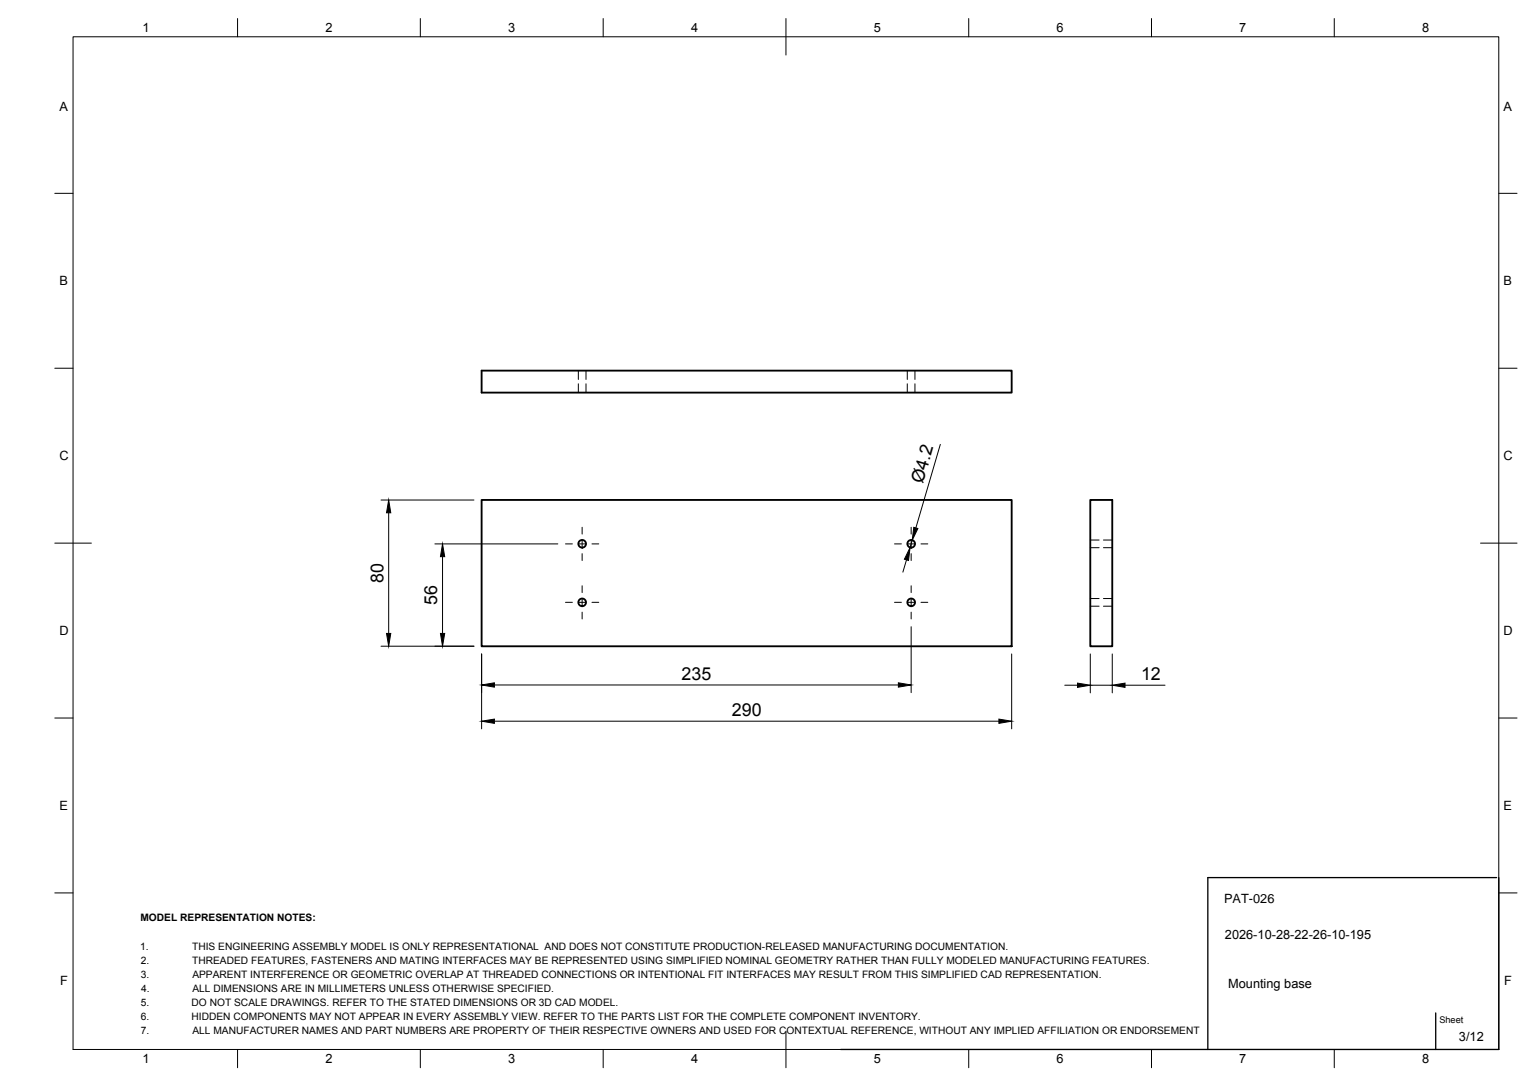
ISO-10303-21;
HEADER;
/* Generated by software containing ST-Developer
 * from STEP Tools, Inc. (www.steptools.com) 
 */

FILE_DESCRIPTION(
/* description */ ('PAT-026'),
/* implementation_level */ '2;1');

FILE_NAME(
/* name */ 'Mounting base.step',
/* time_stamp */ '2026-10-28T22:25:58-07:00',
/* author */ (''),
/* organization */ (''),
/* preprocessor_version */ 'ST-DEVELOPER v20.2',
/* originating_system */ 'Autodesk Translation Framework v15.17.0.0',
/* authorisation */ '');

FILE_SCHEMA (('AUTOMOTIVE_DESIGN { 1 0 10303 214 3 1 1 }'));
ENDSEC;

DATA;
#10=MECHANICAL_DESIGN_GEOMETRIC_PRESENTATION_REPRESENTATION('',(#141),#12343);
#119=SHAPE_REPRESENTATION_RELATIONSHIP('SRR','None',#12396,#130);
#130=ADVANCED_BREP_SHAPE_REPRESENTATION('',(#152),#12331);
#141=STYLED_ITEM('',(#12512),#152);
#152=MANIFOLD_SOLID_BREP('Body1',#7347);
#161=FACE_BOUND('',#965,.T.);
#162=FACE_BOUND('',#966,.T.);
#163=FACE_BOUND('',#967,.T.);
#164=FACE_BOUND('',#968,.T.);
#165=FACE_BOUND('',#970,.T.);
#166=FACE_BOUND('',#971,.T.);
#167=FACE_BOUND('',#972,.T.);
#168=FACE_BOUND('',#973,.T.);
#194=PLANE('',#7496);
#195=PLANE('',#7497);
#196=PLANE('',#7498);
#197=PLANE('',#7499);
#198=PLANE('',#7500);
#199=PLANE('',#7501);
#553=FACE_OUTER_BOUND('',#956,.T.);
#554=FACE_OUTER_BOUND('',#957,.T.);
#555=FACE_OUTER_BOUND('',#958,.T.);
#556=FACE_OUTER_BOUND('',#959,.T.);
#557=FACE_OUTER_BOUND('',#960,.T.);
#558=FACE_OUTER_BOUND('',#961,.T.);
#559=FACE_OUTER_BOUND('',#962,.T.);
#560=FACE_OUTER_BOUND('',#963,.T.);
#561=FACE_OUTER_BOUND('',#964,.T.);
#562=FACE_OUTER_BOUND('',#969,.T.);
#956=EDGE_LOOP('',(#4899,#4900,#4901,#4902));
#957=EDGE_LOOP('',(#4903,#4904,#4905,#4906));
#958=EDGE_LOOP('',(#4907,#4908,#4909,#4910));
#959=EDGE_LOOP('',(#4911,#4912,#4913,#4914));
#960=EDGE_LOOP('',(#4915,#4916,#4917,#4918));
#961=EDGE_LOOP('',(#4919,#4920,#4921,#4922));
#962=EDGE_LOOP('',(#4923,#4924,#4925,#4926));
#963=EDGE_LOOP('',(#4927,#4928,#4929,#4930));
#964=EDGE_LOOP('',(#4931,#4932,#4933,#4934));
#965=EDGE_LOOP('',(#4935));
#966=EDGE_LOOP('',(#4936));
#967=EDGE_LOOP('',(#4937));
#968=EDGE_LOOP('',(#4938));
#969=EDGE_LOOP('',(#4939,#4940,#4941,#4942));
#970=EDGE_LOOP('',(#4943));
#971=EDGE_LOOP('',(#4944));
#972=EDGE_LOOP('',(#4945));
#973=EDGE_LOOP('',(#4946));
#1392=LINE('',#10046,#2264);
#1393=LINE('',#10052,#2265);
#1394=LINE('',#10058,#2266);
#1395=LINE('',#10064,#2267);
#1396=LINE('',#10069,#2268);
#1397=LINE('',#10071,#2269);
#1398=LINE('',#10073,#2270);
#1399=LINE('',#10074,#2271);
#1400=LINE('',#10077,#2272);
#1401=LINE('',#10079,#2273);
#1402=LINE('',#10080,#2274);
#1403=LINE('',#10083,#2275);
#1404=LINE('',#10085,#2276);
#1405=LINE('',#10086,#2277);
#1406=LINE('',#10088,#2278);
#1407=LINE('',#10089,#2279);
#2264=VECTOR('',#8052,0.21);
#2265=VECTOR('',#8059,0.21);
#2266=VECTOR('',#8066,0.21);
#2267=VECTOR('',#8073,0.21);
#2268=VECTOR('',#8078,1.);
#2269=VECTOR('',#8079,1.);
#2270=VECTOR('',#8080,1.);
#2271=VECTOR('',#8081,1.);
#2272=VECTOR('',#8084,1.);
#2273=VECTOR('',#8085,1.);
#2274=VECTOR('',#8086,1.);
#2275=VECTOR('',#8089,1.);
#2276=VECTOR('',#8090,1.);
#2277=VECTOR('',#8091,1.);
#2278=VECTOR('',#8094,1.);
#2279=VECTOR('',#8095,1.);
#3136=CIRCLE('',#7485,0.21);
#3137=CIRCLE('',#7486,0.21);
#3138=CIRCLE('',#7488,0.21);
#3139=CIRCLE('',#7489,0.21);
#3140=CIRCLE('',#7491,0.21);
#3141=CIRCLE('',#7492,0.21);
#3142=CIRCLE('',#7494,0.21);
#3143=CIRCLE('',#7495,0.21);
#3261=VERTEX_POINT('',#10043);
#3262=VERTEX_POINT('',#10045);
#3263=VERTEX_POINT('',#10049);
#3264=VERTEX_POINT('',#10051);
#3265=VERTEX_POINT('',#10055);
#3266=VERTEX_POINT('',#10057);
#3267=VERTEX_POINT('',#10061);
#3268=VERTEX_POINT('',#10063);
#3269=VERTEX_POINT('',#10067);
#3270=VERTEX_POINT('',#10068);
#3271=VERTEX_POINT('',#10070);
#3272=VERTEX_POINT('',#10072);
#3273=VERTEX_POINT('',#10076);
#3274=VERTEX_POINT('',#10078);
#3275=VERTEX_POINT('',#10082);
#3276=VERTEX_POINT('',#10084);
#3893=EDGE_CURVE('',#3261,#3261,#3136,.T.);
#3894=EDGE_CURVE('',#3261,#3262,#1392,.T.);
#3895=EDGE_CURVE('',#3262,#3262,#3137,.T.);
#3896=EDGE_CURVE('',#3263,#3263,#3138,.T.);
#3897=EDGE_CURVE('',#3263,#3264,#1393,.T.);
#3898=EDGE_CURVE('',#3264,#3264,#3139,.T.);
#3899=EDGE_CURVE('',#3265,#3265,#3140,.T.);
#3900=EDGE_CURVE('',#3265,#3266,#1394,.T.);
#3901=EDGE_CURVE('',#3266,#3266,#3141,.T.);
#3902=EDGE_CURVE('',#3267,#3267,#3142,.T.);
#3903=EDGE_CURVE('',#3267,#3268,#1395,.T.);
#3904=EDGE_CURVE('',#3268,#3268,#3143,.T.);
#3905=EDGE_CURVE('',#3269,#3270,#1396,.T.);
#3906=EDGE_CURVE('',#3270,#3271,#1397,.T.);
#3907=EDGE_CURVE('',#3272,#3271,#1398,.T.);
#3908=EDGE_CURVE('',#3269,#3272,#1399,.T.);
#3909=EDGE_CURVE('',#3273,#3269,#1400,.T.);
#3910=EDGE_CURVE('',#3274,#3272,#1401,.T.);
#3911=EDGE_CURVE('',#3273,#3274,#1402,.T.);
#3912=EDGE_CURVE('',#3275,#3273,#1403,.T.);
#3913=EDGE_CURVE('',#3276,#3274,#1404,.T.);
#3914=EDGE_CURVE('',#3275,#3276,#1405,.T.);
#3915=EDGE_CURVE('',#3270,#3275,#1406,.T.);
#3916=EDGE_CURVE('',#3271,#3276,#1407,.T.);
#4899=ORIENTED_EDGE('',*,*,#3893,.F.);
#4900=ORIENTED_EDGE('',*,*,#3894,.T.);
#4901=ORIENTED_EDGE('',*,*,#3895,.F.);
#4902=ORIENTED_EDGE('',*,*,#3894,.F.);
#4903=ORIENTED_EDGE('',*,*,#3896,.F.);
#4904=ORIENTED_EDGE('',*,*,#3897,.T.);
#4905=ORIENTED_EDGE('',*,*,#3898,.F.);
#4906=ORIENTED_EDGE('',*,*,#3897,.F.);
#4907=ORIENTED_EDGE('',*,*,#3899,.F.);
#4908=ORIENTED_EDGE('',*,*,#3900,.T.);
#4909=ORIENTED_EDGE('',*,*,#3901,.F.);
#4910=ORIENTED_EDGE('',*,*,#3900,.F.);
#4911=ORIENTED_EDGE('',*,*,#3902,.F.);
#4912=ORIENTED_EDGE('',*,*,#3903,.T.);
#4913=ORIENTED_EDGE('',*,*,#3904,.F.);
#4914=ORIENTED_EDGE('',*,*,#3903,.F.);
#4915=ORIENTED_EDGE('',*,*,#3905,.T.);
#4916=ORIENTED_EDGE('',*,*,#3906,.T.);
#4917=ORIENTED_EDGE('',*,*,#3907,.F.);
#4918=ORIENTED_EDGE('',*,*,#3908,.F.);
#4919=ORIENTED_EDGE('',*,*,#3909,.T.);
#4920=ORIENTED_EDGE('',*,*,#3908,.T.);
#4921=ORIENTED_EDGE('',*,*,#3910,.F.);
#4922=ORIENTED_EDGE('',*,*,#3911,.F.);
#4923=ORIENTED_EDGE('',*,*,#3912,.T.);
#4924=ORIENTED_EDGE('',*,*,#3911,.T.);
#4925=ORIENTED_EDGE('',*,*,#3913,.F.);
#4926=ORIENTED_EDGE('',*,*,#3914,.F.);
#4927=ORIENTED_EDGE('',*,*,#3915,.T.);
#4928=ORIENTED_EDGE('',*,*,#3914,.T.);
#4929=ORIENTED_EDGE('',*,*,#3916,.F.);
#4930=ORIENTED_EDGE('',*,*,#3906,.F.);
#4931=ORIENTED_EDGE('',*,*,#3916,.T.);
#4932=ORIENTED_EDGE('',*,*,#3913,.T.);
#4933=ORIENTED_EDGE('',*,*,#3910,.T.);
#4934=ORIENTED_EDGE('',*,*,#3907,.T.);
#4935=ORIENTED_EDGE('',*,*,#3895,.T.);
#4936=ORIENTED_EDGE('',*,*,#3898,.T.);
#4937=ORIENTED_EDGE('',*,*,#3901,.T.);
#4938=ORIENTED_EDGE('',*,*,#3904,.T.);
#4939=ORIENTED_EDGE('',*,*,#3915,.F.);
#4940=ORIENTED_EDGE('',*,*,#3905,.F.);
#4941=ORIENTED_EDGE('',*,*,#3909,.F.);
#4942=ORIENTED_EDGE('',*,*,#3912,.F.);
#4943=ORIENTED_EDGE('',*,*,#3893,.T.);
#4944=ORIENTED_EDGE('',*,*,#3896,.T.);
#4945=ORIENTED_EDGE('',*,*,#3899,.T.);
#4946=ORIENTED_EDGE('',*,*,#3902,.T.);
#6911=CYLINDRICAL_SURFACE('',#7484,0.21);
#6912=CYLINDRICAL_SURFACE('',#7487,0.21);
#6913=CYLINDRICAL_SURFACE('',#7490,0.21);
#6914=CYLINDRICAL_SURFACE('',#7493,0.21);
#6944=ADVANCED_FACE('',(#553),#6911,.F.);
#6945=ADVANCED_FACE('',(#554),#6912,.F.);
#6946=ADVANCED_FACE('',(#555),#6913,.F.);
#6947=ADVANCED_FACE('',(#556),#6914,.F.);
#6948=ADVANCED_FACE('',(#557),#194,.T.);
#6949=ADVANCED_FACE('',(#558),#195,.T.);
#6950=ADVANCED_FACE('',(#559),#196,.T.);
#6951=ADVANCED_FACE('',(#560),#197,.T.);
#6952=ADVANCED_FACE('',(#561,#161,#162,#163,#164),#198,.T.);
#6953=ADVANCED_FACE('',(#562,#165,#166,#167,#168),#199,.F.);
#7347=CLOSED_SHELL('',(#6944,#6945,#6946,#6947,#6948,#6949,#6950,#6951,
#6952,#6953));
#7483=AXIS2_PLACEMENT_3D('',#10041,#8046,#8047);
#7484=AXIS2_PLACEMENT_3D('',#10042,#8048,#8049);
#7485=AXIS2_PLACEMENT_3D('',#10044,#8050,#8051);
#7486=AXIS2_PLACEMENT_3D('',#10047,#8053,#8054);
#7487=AXIS2_PLACEMENT_3D('',#10048,#8055,#8056);
#7488=AXIS2_PLACEMENT_3D('',#10050,#8057,#8058);
#7489=AXIS2_PLACEMENT_3D('',#10053,#8060,#8061);
#7490=AXIS2_PLACEMENT_3D('',#10054,#8062,#8063);
#7491=AXIS2_PLACEMENT_3D('',#10056,#8064,#8065);
#7492=AXIS2_PLACEMENT_3D('',#10059,#8067,#8068);
#7493=AXIS2_PLACEMENT_3D('',#10060,#8069,#8070);
#7494=AXIS2_PLACEMENT_3D('',#10062,#8071,#8072);
#7495=AXIS2_PLACEMENT_3D('',#10065,#8074,#8075);
#7496=AXIS2_PLACEMENT_3D('',#10066,#8076,#8077);
#7497=AXIS2_PLACEMENT_3D('',#10075,#8082,#8083);
#7498=AXIS2_PLACEMENT_3D('',#10081,#8087,#8088);
#7499=AXIS2_PLACEMENT_3D('',#10087,#8092,#8093);
#7500=AXIS2_PLACEMENT_3D('',#10090,#8096,#8097);
#7501=AXIS2_PLACEMENT_3D('',#10091,#8098,#8099);
#8046=DIRECTION('axis',(0.,0.,1.));
#8047=DIRECTION('refdir',(1.,0.,0.));
#8048=DIRECTION('center_axis',(0.,0.,1.));
#8049=DIRECTION('ref_axis',(1.,0.,0.));
#8050=DIRECTION('center_axis',(0.,0.,1.));
#8051=DIRECTION('ref_axis',(1.,0.,0.));
#8052=DIRECTION('',(0.,0.,1.));
#8053=DIRECTION('center_axis',(0.,0.,-1.));
#8054=DIRECTION('ref_axis',(1.,0.,0.));
#8055=DIRECTION('center_axis',(0.,0.,1.));
#8056=DIRECTION('ref_axis',(1.,0.,0.));
#8057=DIRECTION('center_axis',(0.,0.,1.));
#8058=DIRECTION('ref_axis',(1.,0.,0.));
#8059=DIRECTION('',(0.,0.,1.));
#8060=DIRECTION('center_axis',(0.,0.,-1.));
#8061=DIRECTION('ref_axis',(1.,0.,0.));
#8062=DIRECTION('center_axis',(0.,0.,1.));
#8063=DIRECTION('ref_axis',(1.,0.,0.));
#8064=DIRECTION('center_axis',(0.,0.,1.));
#8065=DIRECTION('ref_axis',(1.,0.,0.));
#8066=DIRECTION('',(0.,0.,1.));
#8067=DIRECTION('center_axis',(0.,0.,-1.));
#8068=DIRECTION('ref_axis',(1.,0.,0.));
#8069=DIRECTION('center_axis',(0.,0.,1.));
#8070=DIRECTION('ref_axis',(1.,0.,0.));
#8071=DIRECTION('center_axis',(0.,0.,1.));
#8072=DIRECTION('ref_axis',(1.,0.,0.));
#8073=DIRECTION('',(0.,0.,1.));
#8074=DIRECTION('center_axis',(0.,0.,-1.));
#8075=DIRECTION('ref_axis',(1.,0.,0.));
#8076=DIRECTION('center_axis',(0.,1.,0.));
#8077=DIRECTION('ref_axis',(-1.,0.,0.));
#8078=DIRECTION('',(-1.,0.,0.));
#8079=DIRECTION('',(0.,0.,1.));
#8080=DIRECTION('',(-1.,0.,0.));
#8081=DIRECTION('',(0.,0.,1.));
#8082=DIRECTION('center_axis',(1.,0.,0.));
#8083=DIRECTION('ref_axis',(0.,1.,0.));
#8084=DIRECTION('',(0.,1.,0.));
#8085=DIRECTION('',(0.,1.,0.));
#8086=DIRECTION('',(0.,0.,1.));
#8087=DIRECTION('center_axis',(0.,-1.,0.));
#8088=DIRECTION('ref_axis',(1.,0.,0.));
#8089=DIRECTION('',(1.,0.,0.));
#8090=DIRECTION('',(1.,0.,0.));
#8091=DIRECTION('',(0.,0.,1.));
#8092=DIRECTION('center_axis',(-1.,0.,0.));
#8093=DIRECTION('ref_axis',(0.,-1.,0.));
#8094=DIRECTION('',(0.,-1.,0.));
#8095=DIRECTION('',(0.,-1.,0.));
#8096=DIRECTION('center_axis',(0.,0.,1.));
#8097=DIRECTION('ref_axis',(1.,0.,0.));
#8098=DIRECTION('center_axis',(0.,0.,1.));
#8099=DIRECTION('ref_axis',(1.,0.,0.));
#10041=CARTESIAN_POINT('',(0.,0.,0.));
#10042=CARTESIAN_POINT('Origin',(1.6,-9.,-0.1));
#10043=CARTESIAN_POINT('',(1.39,-9.,0.));
#10044=CARTESIAN_POINT('Origin',(1.6,-9.,0.));
#10045=CARTESIAN_POINT('',(1.39,-9.,1.2));
#10046=CARTESIAN_POINT('',(1.39,-9.,-0.1));
#10047=CARTESIAN_POINT('Origin',(1.6,-9.,1.2));
#10048=CARTESIAN_POINT('Origin',(-1.6,9.,-0.1));
#10049=CARTESIAN_POINT('',(-1.81,9.,0.));
#10050=CARTESIAN_POINT('Origin',(-1.6,9.,0.));
#10051=CARTESIAN_POINT('',(-1.81,9.,1.2));
#10052=CARTESIAN_POINT('',(-1.81,9.,-0.1));
#10053=CARTESIAN_POINT('Origin',(-1.6,9.,1.2));
#10054=CARTESIAN_POINT('Origin',(-1.6,-9.,-0.1));
#10055=CARTESIAN_POINT('',(-1.81,-9.,0.));
#10056=CARTESIAN_POINT('Origin',(-1.6,-9.,0.));
#10057=CARTESIAN_POINT('',(-1.81,-9.,1.2));
#10058=CARTESIAN_POINT('',(-1.81,-9.,-0.1));
#10059=CARTESIAN_POINT('Origin',(-1.6,-9.,1.2));
#10060=CARTESIAN_POINT('Origin',(1.6,9.,-0.1));
#10061=CARTESIAN_POINT('',(1.39,9.,0.));
#10062=CARTESIAN_POINT('Origin',(1.6,9.,0.));
#10063=CARTESIAN_POINT('',(1.39,9.,1.2));
#10064=CARTESIAN_POINT('',(1.39,9.,-0.1));
#10065=CARTESIAN_POINT('Origin',(1.6,9.,1.2));
#10066=CARTESIAN_POINT('Origin',(4.,14.5,0.));
#10067=CARTESIAN_POINT('',(4.,14.5,0.));
#10068=CARTESIAN_POINT('',(-4.,14.5,0.));
#10069=CARTESIAN_POINT('',(4.,14.5,0.));
#10070=CARTESIAN_POINT('',(-4.,14.5,1.2));
#10071=CARTESIAN_POINT('',(-4.,14.5,0.));
#10072=CARTESIAN_POINT('',(4.,14.5,1.2));
#10073=CARTESIAN_POINT('',(4.,14.5,1.2));
#10074=CARTESIAN_POINT('',(4.,14.5,0.));
#10075=CARTESIAN_POINT('Origin',(4.,-14.5,0.));
#10076=CARTESIAN_POINT('',(4.,-14.5,0.));
#10077=CARTESIAN_POINT('',(4.,-14.5,0.));
#10078=CARTESIAN_POINT('',(4.,-14.5,1.2));
#10079=CARTESIAN_POINT('',(4.,-14.5,1.2));
#10080=CARTESIAN_POINT('',(4.,-14.5,0.));
#10081=CARTESIAN_POINT('Origin',(-4.,-14.5,0.));
#10082=CARTESIAN_POINT('',(-4.,-14.5,0.));
#10083=CARTESIAN_POINT('',(-4.,-14.5,0.));
#10084=CARTESIAN_POINT('',(-4.,-14.5,1.2));
#10085=CARTESIAN_POINT('',(-4.,-14.5,1.2));
#10086=CARTESIAN_POINT('',(-4.,-14.5,0.));
#10087=CARTESIAN_POINT('Origin',(-4.,14.5,0.));
#10088=CARTESIAN_POINT('',(-4.,14.5,0.));
#10089=CARTESIAN_POINT('',(-4.,14.5,1.2));
#10090=CARTESIAN_POINT('Origin',(0.,0.,1.2));
#10091=CARTESIAN_POINT('Origin',(0.,0.,0.));
#12317=UNCERTAINTY_MEASURE_WITH_UNIT(LENGTH_MEASURE(0.001),#12344,
'DISTANCE_ACCURACY_VALUE',
'Maximum model space distance between geometric entities at asserted c
onnectivities');
#12329=UNCERTAINTY_MEASURE_WITH_UNIT(LENGTH_MEASURE(0.001),#12344,
'DISTANCE_ACCURACY_VALUE',
'Maximum model space distance between geometric entities at asserted c
onnectivities');
#12331=(
GEOMETRIC_REPRESENTATION_CONTEXT(3)
GLOBAL_UNCERTAINTY_ASSIGNED_CONTEXT((#12317))
GLOBAL_UNIT_ASSIGNED_CONTEXT((#12344,#12346,#12347))
REPRESENTATION_CONTEXT('','3D')
);
#12343=(
GEOMETRIC_REPRESENTATION_CONTEXT(3)
GLOBAL_UNCERTAINTY_ASSIGNED_CONTEXT((#12329))
GLOBAL_UNIT_ASSIGNED_CONTEXT((#12344,#12346,#12347))
REPRESENTATION_CONTEXT('','3D')
);
#12344=(
LENGTH_UNIT()
NAMED_UNIT(*)
SI_UNIT(.CENTI.,.METRE.)
);
#12346=(
NAMED_UNIT(*)
PLANE_ANGLE_UNIT()
SI_UNIT($,.RADIAN.)
);
#12347=(
NAMED_UNIT(*)
SI_UNIT($,.STERADIAN.)
SOLID_ANGLE_UNIT()
);
#12349=SHAPE_DEFINITION_REPRESENTATION(#12362,#12396);
#12362=PRODUCT_DEFINITION_SHAPE('',$,#12410);
#12396=SHAPE_REPRESENTATION('',(#7483),#12331);
#12408=PRODUCT_DEFINITION_CONTEXT('part definition',#12449,'design');
#12410=PRODUCT_DEFINITION('Mounting base','Mounting base',#12423,
#12408);
#12423=PRODUCT_DEFINITION_FORMATION('',$,#12452);
#12449=APPLICATION_CONTEXT(
'Core Data for Automotive Mechanical Design Process');
#12450=PRODUCT_CONTEXT('part definition',#12449,'mechanical');
#12452=PRODUCT('Mounting base','Mounting base',
'Mounting base',(#12450));
#12506=COLOUR_RGB('Dark Blue',0.08,0.2,0.34);
#12507=FILL_AREA_STYLE_COLOUR('',#12506);
#12508=FILL_AREA_STYLE('',(#12507));
#12509=SURFACE_STYLE_FILL_AREA(#12508);
#12510=SURFACE_SIDE_STYLE('',(#12509));
#12511=SURFACE_STYLE_USAGE(.BOTH.,#12510);
#12512=PRESENTATION_STYLE_ASSIGNMENT((#12511));
ENDSEC;
END-ISO-10303-21;
